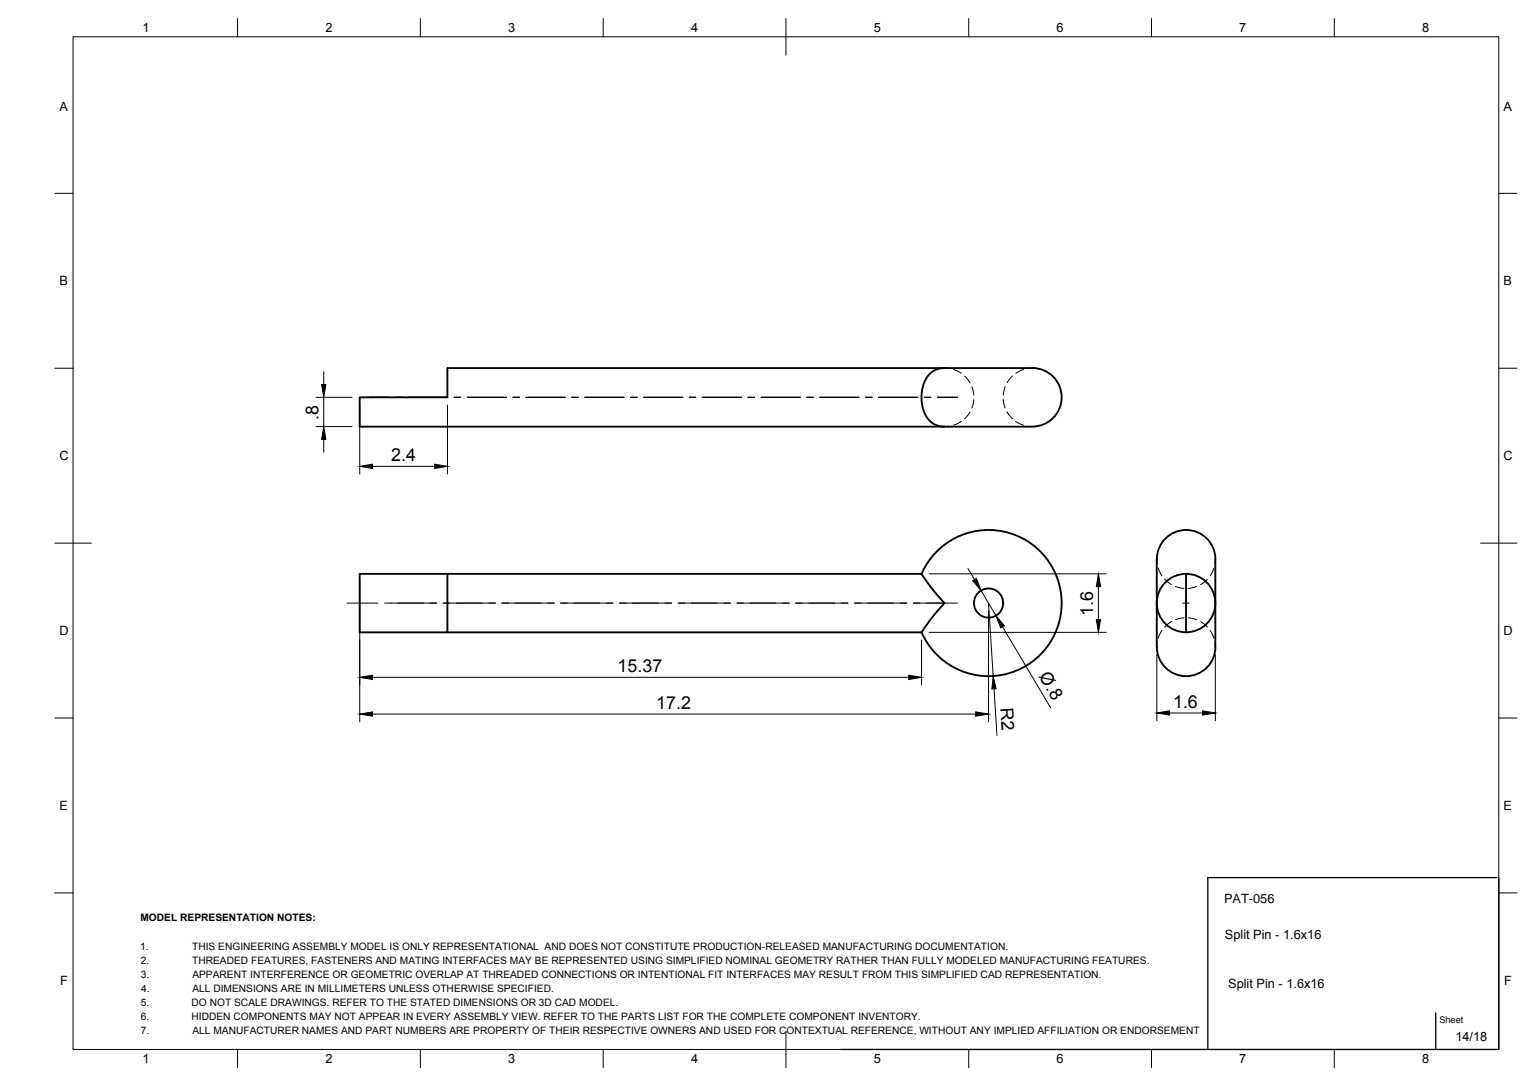
ISO-10303-21;
HEADER;
/* Generated by software containing ST-Developer
 * from STEP Tools, Inc. (www.steptools.com) 
 */

FILE_DESCRIPTION(
/* description */ ('Hook toggle clamp'),
/* implementation_level */ '2;1');

FILE_NAME(
/* name */ 'Split Pin - 1.6x16.step',
/* time_stamp */ '2026-10-27T21:56:56-07:00',
/* author */ (''),
/* organization */ (''),
/* preprocessor_version */ 'ST-DEVELOPER v20.2',
/* originating_system */ 'Autodesk Translation Framework v15.17.0.0',
/* authorisation */ '');

FILE_SCHEMA (('AUTOMOTIVE_DESIGN { 1 0 10303 214 3 1 1 }'));
ENDSEC;

DATA;
#10=MECHANICAL_DESIGN_GEOMETRIC_PRESENTATION_REPRESENTATION('',(#202),#5458);
#11=TOROIDAL_SURFACE('',#3441,0.12,0.08);
#17=B_SPLINE_CURVE_WITH_KNOTS('',3,(#5209,#5210,#5211,#5212,#5213,#5214,
#5215,#5216,#5217,#5218,#5219,#5220,#5221,#5222,#5223,#5224,#5225,#5226,
#5227,#5228,#5229,#5230,#5231,#5232,#5233,#5234),.UNSPECIFIED.,.F.,.F.,
(4,2,2,2,2,2,2,2,2,2,2,2,4),(-0.00054581412719389,0.,0.0281583564005144,
0.0618496465371181,0.0905865724114538,0.120694112793616,0.144966158459363,
0.16923820412511,0.199345744507272,0.228082670381608,0.261773960518212,
0.289932316918681,0.290478131045882),.UNSPECIFIED.);
#18=B_SPLINE_CURVE_WITH_KNOTS('',3,(#5235,#5236,#5237,#5238,#5239,#5240,
#5241,#5242,#5243,#5244,#5245,#5246,#5247,#5248,#5249,#5250,#5251,#5252,
#5253,#5254,#5255,#5256,#5257,#5258,#5259,#5260),.UNSPECIFIED.,.F.,.F.,
(4,2,2,2,2,2,2,2,2,2,2,2,4),(-0.000545814127196571,0.,0.0281583564006391,
0.0618496465374156,0.0905865724118984,0.120694112794215,0.144966158460086,
0.169238204125958,0.199345744508275,0.228082670382758,0.261773960519534,
0.289932316920171,0.29047813104737),.UNSPECIFIED.);
#168=SHAPE_REPRESENTATION_RELATIONSHIP('SRR','None',#5552,#185);
#185=ADVANCED_BREP_SHAPE_REPRESENTATION('',(#218),#5454);
#202=STYLED_ITEM('',(#5717),#218);
#218=MANIFOLD_SOLID_BREP('Body1',#2984);
#273=FACE_BOUND('',#766,.T.);
#378=PLANE('',#3444);
#379=PLANE('',#3446);
#380=PLANE('',#3450);
#541=FACE_OUTER_BOUND('',#765,.T.);
#542=FACE_OUTER_BOUND('',#767,.T.);
#543=FACE_OUTER_BOUND('',#768,.T.);
#544=FACE_OUTER_BOUND('',#769,.T.);
#545=FACE_OUTER_BOUND('',#770,.T.);
#765=EDGE_LOOP('',(#2645,#2646,#2647,#2648));
#766=EDGE_LOOP('',(#2649,#2650));
#767=EDGE_LOOP('',(#2651,#2652));
#768=EDGE_LOOP('',(#2653,#2654,#2655,#2656));
#769=EDGE_LOOP('',(#2657,#2658,#2659,#2660,#2661,#2662,#2663,#2664,#2665));
#770=EDGE_LOOP('',(#2666,#2667,#2668));
#1014=LINE('',#5265,#1251);
#1015=LINE('',#5268,#1252);
#1016=LINE('',#5270,#1253);
#1017=LINE('',#5271,#1254);
#1018=LINE('',#5275,#1255);
#1251=VECTOR('',#4270,1.);
#1252=VECTOR('',#4273,1.);
#1253=VECTOR('',#4274,1.);
#1254=VECTOR('',#4275,1.);
#1255=VECTOR('',#4280,0.08);
#1362=CIRCLE('',#3442,0.08);
#1363=CIRCLE('',#3443,0.04);
#1364=CIRCLE('',#3445,0.08);
#1365=CIRCLE('',#3448,0.08);
#1366=CIRCLE('',#3449,0.08);
#1593=VERTEX_POINT('',#5204);
#1594=VERTEX_POINT('',#5207);
#1595=VERTEX_POINT('',#5208);
#1596=VERTEX_POINT('',#5262);
#1597=VERTEX_POINT('',#5263);
#1598=VERTEX_POINT('',#5267);
#1599=VERTEX_POINT('',#5269);
#1600=VERTEX_POINT('',#5273);
#1949=EDGE_CURVE('',#1593,#1593,#1362,.T.);
#1950=EDGE_CURVE('',#1593,#1593,#1363,.T.);
#1951=EDGE_CURVE('',#1594,#1595,#17,.T.);
#1952=EDGE_CURVE('',#1595,#1594,#18,.T.);
#1953=EDGE_CURVE('',#1596,#1597,#1364,.T.);
#1954=EDGE_CURVE('',#1596,#1597,#1014,.T.);
#1955=EDGE_CURVE('',#1597,#1598,#1015,.T.);
#1956=EDGE_CURVE('',#1599,#1598,#1016,.T.);
#1957=EDGE_CURVE('',#1596,#1599,#1017,.T.);
#1958=EDGE_CURVE('',#1600,#1599,#1365,.T.);
#1959=EDGE_CURVE('',#1600,#1595,#1018,.T.);
#1960=EDGE_CURVE('',#1598,#1600,#1366,.T.);
#2645=ORIENTED_EDGE('',*,*,#1949,.F.);
#2646=ORIENTED_EDGE('',*,*,#1950,.T.);
#2647=ORIENTED_EDGE('',*,*,#1949,.T.);
#2648=ORIENTED_EDGE('',*,*,#1950,.F.);
#2649=ORIENTED_EDGE('',*,*,#1951,.F.);
#2650=ORIENTED_EDGE('',*,*,#1952,.F.);
#2651=ORIENTED_EDGE('',*,*,#1953,.T.);
#2652=ORIENTED_EDGE('',*,*,#1954,.F.);
#2653=ORIENTED_EDGE('',*,*,#1954,.T.);
#2654=ORIENTED_EDGE('',*,*,#1955,.T.);
#2655=ORIENTED_EDGE('',*,*,#1956,.F.);
#2656=ORIENTED_EDGE('',*,*,#1957,.F.);
#2657=ORIENTED_EDGE('',*,*,#1953,.F.);
#2658=ORIENTED_EDGE('',*,*,#1957,.T.);
#2659=ORIENTED_EDGE('',*,*,#1958,.F.);
#2660=ORIENTED_EDGE('',*,*,#1959,.T.);
#2661=ORIENTED_EDGE('',*,*,#1952,.T.);
#2662=ORIENTED_EDGE('',*,*,#1951,.T.);
#2663=ORIENTED_EDGE('',*,*,#1959,.F.);
#2664=ORIENTED_EDGE('',*,*,#1960,.F.);
#2665=ORIENTED_EDGE('',*,*,#1955,.F.);
#2666=ORIENTED_EDGE('',*,*,#1960,.T.);
#2667=ORIENTED_EDGE('',*,*,#1958,.T.);
#2668=ORIENTED_EDGE('',*,*,#1956,.T.);
#2791=CYLINDRICAL_SURFACE('',#3447,0.08);
#2945=ADVANCED_FACE('',(#541,#273),#11,.T.);
#2946=ADVANCED_FACE('',(#542),#378,.F.);
#2947=ADVANCED_FACE('',(#543),#379,.T.);
#2948=ADVANCED_FACE('',(#544),#2791,.T.);
#2949=ADVANCED_FACE('',(#545),#380,.F.);
#2984=CLOSED_SHELL('',(#2945,#2946,#2947,#2948,#2949));
#3440=AXIS2_PLACEMENT_3D('',#5202,#4258,#4259);
#3441=AXIS2_PLACEMENT_3D('',#5203,#4260,#4261);
#3442=AXIS2_PLACEMENT_3D('',#5205,#4262,#4263);
#3443=AXIS2_PLACEMENT_3D('',#5206,#4264,#4265);
#3444=AXIS2_PLACEMENT_3D('',#5261,#4266,#4267);
#3445=AXIS2_PLACEMENT_3D('',#5264,#4268,#4269);
#3446=AXIS2_PLACEMENT_3D('',#5266,#4271,#4272);
#3447=AXIS2_PLACEMENT_3D('',#5272,#4276,#4277);
#3448=AXIS2_PLACEMENT_3D('',#5274,#4278,#4279);
#3449=AXIS2_PLACEMENT_3D('',#5276,#4281,#4282);
#3450=AXIS2_PLACEMENT_3D('',#5277,#4283,#4284);
#4258=DIRECTION('axis',(0.,0.,1.));
#4259=DIRECTION('refdir',(1.,0.,0.));
#4260=DIRECTION('center_axis',(-1.,0.,0.));
#4261=DIRECTION('ref_axis',(0.,0.,1.));
#4262=DIRECTION('center_axis',(0.,-1.,1.38777878078145E-16));
#4263=DIRECTION('ref_axis',(0.,-1.38777878078145E-16,-1.));
#4264=DIRECTION('center_axis',(1.,0.,0.));
#4265=DIRECTION('ref_axis',(0.,0.,1.));
#4266=DIRECTION('center_axis',(0.,1.,0.));
#4267=DIRECTION('ref_axis',(1.,0.,0.));
#4268=DIRECTION('center_axis',(0.,-1.,0.));
#4269=DIRECTION('ref_axis',(1.,0.,0.));
#4270=DIRECTION('',(0.,0.,1.));
#4271=DIRECTION('center_axis',(1.,0.,0.));
#4272=DIRECTION('ref_axis',(0.,0.,1.));
#4273=DIRECTION('',(0.,-1.,0.));
#4274=DIRECTION('',(0.,0.,1.));
#4275=DIRECTION('',(0.,-1.,0.));
#4276=DIRECTION('center_axis',(0.,-1.,0.));
#4277=DIRECTION('ref_axis',(1.,0.,0.));
#4278=DIRECTION('center_axis',(0.,-1.,0.));
#4279=DIRECTION('ref_axis',(1.,0.,0.));
#4280=DIRECTION('',(0.,1.,0.));
#4281=DIRECTION('center_axis',(0.,-1.,0.));
#4282=DIRECTION('ref_axis',(1.,0.,0.));
#4283=DIRECTION('center_axis',(0.,1.,0.));
#4284=DIRECTION('ref_axis',(1.,0.,0.));
#5202=CARTESIAN_POINT('',(0.,0.,0.));
#5203=CARTESIAN_POINT('Origin',(0.,0.12,0.));
#5204=CARTESIAN_POINT('',(-9.79717439317883E-18,0.12,-0.04));
#5205=CARTESIAN_POINT('Origin',(0.,0.12,-0.12));
#5206=CARTESIAN_POINT('Origin',(9.79717439317883E-18,0.12,0.));
#5207=CARTESIAN_POINT('',(0.08,-4.89858719658941E-18,7.34788079488412E-18));
#5208=CARTESIAN_POINT('',(-0.08,-4.89858719658941E-18,7.34788079488412E-18));
#5209=CARTESIAN_POINT('Ctrl Pts',(0.08,-4.89858719658941E-18,7.34788079488412E-18));
#5210=CARTESIAN_POINT('Ctrl Pts',(0.08,-0.00012864962353541,0.000128649623535413));
#5211=CARTESIAN_POINT('Ctrl Pts',(0.0799996896739287,-0.00025719571182076,
0.000257402596003253));
#5212=CARTESIAN_POINT('Ctrl Pts',(0.0799669711262291,-0.00701193164572964,
0.00703384588894362));
#5213=CARTESIAN_POINT('Ctrl Pts',(0.0791054994909294,-0.0133457972655825,
0.0139383126556792));
#5214=CARTESIAN_POINT('Ctrl Pts',(0.0749700088488058,-0.0265076530862524,
0.0292212026164895));
#5215=CARTESIAN_POINT('Ctrl Pts',(0.0712702072865517,-0.0331317062461458,
0.0375603420117568));
#5216=CARTESIAN_POINT('Ctrl Pts',(0.0612858949407667,-0.0440683985740427,
0.0520545604187517));
#5217=CARTESIAN_POINT('Ctrl Pts',(0.0555090276731744,-0.0485199197794574,
0.0582717815295611));
#5218=CARTESIAN_POINT('Ctrl Pts',(0.0412398082144208,-0.0561090538733877,
0.0691638397919718));
#5219=CARTESIAN_POINT('Ctrl Pts',(0.0327878980890048,-0.059089642483296,
0.0736229049587921));
#5220=CARTESIAN_POINT('Ctrl Pts',(0.0159233027310102,-0.0625179833270725,
0.0787936360751706));
#5221=CARTESIAN_POINT('Ctrl Pts',(0.00801661414593076,-0.0633030277982336,
0.08));
#5222=CARTESIAN_POINT('Ctrl Pts',(-0.00801661414593074,-0.0633030277982336,
0.08));
#5223=CARTESIAN_POINT('Ctrl Pts',(-0.0159233027310102,-0.0625179833270726,
0.0787936360751706));
#5224=CARTESIAN_POINT('Ctrl Pts',(-0.0327878980890049,-0.059089642483296,
0.0736229049587921));
#5225=CARTESIAN_POINT('Ctrl Pts',(-0.0412398082144209,-0.0561090538733877,
0.0691638397919717));
#5226=CARTESIAN_POINT('Ctrl Pts',(-0.0555090276731744,-0.0485199197794574,
0.0582717815295611));
#5227=CARTESIAN_POINT('Ctrl Pts',(-0.0612858949407667,-0.0440683985740427,
0.0520545604187517));
#5228=CARTESIAN_POINT('Ctrl Pts',(-0.0712702072865517,-0.0331317062461458,
0.0375603420117568));
#5229=CARTESIAN_POINT('Ctrl Pts',(-0.0749700088488058,-0.0265076530862524,
0.0292212026164895));
#5230=CARTESIAN_POINT('Ctrl Pts',(-0.0791054994909264,-0.0133457972655921,
0.0139383126556903));
#5231=CARTESIAN_POINT('Ctrl Pts',(-0.0799669711262287,-0.00701193164579759,
0.0070338458890125));
#5232=CARTESIAN_POINT('Ctrl Pts',(-0.0799996896739287,-0.000257195711817665,
0.000257402596000083));
#5233=CARTESIAN_POINT('Ctrl Pts',(-0.08,-0.000128649623538514,0.000128649623538516));
#5234=CARTESIAN_POINT('Ctrl Pts',(-0.08,-4.89858719658941E-18,7.34788079488412E-18));
#5235=CARTESIAN_POINT('Ctrl Pts',(-0.08,-4.89858719658941E-18,7.34788079488412E-18));
#5236=CARTESIAN_POINT('Ctrl Pts',(-0.08,-0.000128649623536042,-0.00012864962353603));
#5237=CARTESIAN_POINT('Ctrl Pts',(-0.0799996896739287,-0.000257195711820127,
-0.000257402596002604));
#5238=CARTESIAN_POINT('Ctrl Pts',(-0.0799669711262289,-0.0070119316457589,
-0.00703384588897312));
#5239=CARTESIAN_POINT('Ctrl Pts',(-0.0791054994909281,-0.0133457972655867,
-0.0139383126556841));
#5240=CARTESIAN_POINT('Ctrl Pts',(-0.0749700088488058,-0.0265076530862525,
-0.0292212026164896));
#5241=CARTESIAN_POINT('Ctrl Pts',(-0.0712702072865516,-0.0331317062461459,
-0.0375603420117568));
#5242=CARTESIAN_POINT('Ctrl Pts',(-0.0612858949407667,-0.0440683985740427,
-0.0520545604187517));
#5243=CARTESIAN_POINT('Ctrl Pts',(-0.0555090276731744,-0.0485199197794574,
-0.0582717815295611));
#5244=CARTESIAN_POINT('Ctrl Pts',(-0.0412398082144209,-0.0561090538733877,
-0.0691638397919717));
#5245=CARTESIAN_POINT('Ctrl Pts',(-0.0327878980890049,-0.059089642483296,
-0.0736229049587921));
#5246=CARTESIAN_POINT('Ctrl Pts',(-0.0159233027310101,-0.0625179833270725,
-0.0787936360751706));
#5247=CARTESIAN_POINT('Ctrl Pts',(-0.00801661414593069,-0.0633030277982336,
-0.08));
#5248=CARTESIAN_POINT('Ctrl Pts',(0.0080166141459307,-0.0633030277982336,
-0.08));
#5249=CARTESIAN_POINT('Ctrl Pts',(0.0159233027310101,-0.0625179833270725,
-0.0787936360751706));
#5250=CARTESIAN_POINT('Ctrl Pts',(0.0327878980890049,-0.0590896424832959,
-0.0736229049587921));
#5251=CARTESIAN_POINT('Ctrl Pts',(0.0412398082144209,-0.0561090538733877,
-0.0691638397919717));
#5252=CARTESIAN_POINT('Ctrl Pts',(0.0555090276731744,-0.0485199197794574,
-0.0582717815295611));
#5253=CARTESIAN_POINT('Ctrl Pts',(0.0612858949407666,-0.0440683985740428,
-0.0520545604187518));
#5254=CARTESIAN_POINT('Ctrl Pts',(0.0712702072865517,-0.0331317062461458,
-0.0375603420117568));
#5255=CARTESIAN_POINT('Ctrl Pts',(0.0749700088488058,-0.0265076530862524,
-0.0292212026164895));
#5256=CARTESIAN_POINT('Ctrl Pts',(0.079105499490928,-0.013345797265587,
-0.0139383126556845));
#5257=CARTESIAN_POINT('Ctrl Pts',(0.0799669711262289,-0.00701193164576148,
-0.00703384588897579));
#5258=CARTESIAN_POINT('Ctrl Pts',(0.0799996896739287,-0.000257195711819584,
-0.000257402596002039));
#5259=CARTESIAN_POINT('Ctrl Pts',(0.08,-0.000128649623536605,-0.000128649623536593));
#5260=CARTESIAN_POINT('Ctrl Pts',(0.08,-4.89858719658941E-18,7.34788079488412E-18));
#5261=CARTESIAN_POINT('Origin',(0.04,-1.36,0.));
#5262=CARTESIAN_POINT('',(0.,-1.36,-0.08));
#5263=CARTESIAN_POINT('',(0.,-1.36,0.08));
#5264=CARTESIAN_POINT('Origin',(0.,-1.36,0.));
#5265=CARTESIAN_POINT('',(0.,-1.36,-0.04));
#5266=CARTESIAN_POINT('Origin',(0.,0.,-0.08));
#5267=CARTESIAN_POINT('',(0.,-1.6,0.08));
#5268=CARTESIAN_POINT('',(0.,0.,0.08));
#5269=CARTESIAN_POINT('',(0.,-1.6,-0.08));
#5270=CARTESIAN_POINT('',(0.,-1.6,-0.09));
#5271=CARTESIAN_POINT('',(0.,0.,-0.08));
#5272=CARTESIAN_POINT('Origin',(0.,0.,0.));
#5273=CARTESIAN_POINT('',(-0.08,-1.6,-9.79717439317883E-18));
#5274=CARTESIAN_POINT('Origin',(0.,-1.6,0.));
#5275=CARTESIAN_POINT('',(-0.08,0.,-9.79717439317883E-18));
#5276=CARTESIAN_POINT('Origin',(0.,-1.6,0.));
#5277=CARTESIAN_POINT('Origin',(-0.04,-1.6,0.));
#5431=UNCERTAINTY_MEASURE_WITH_UNIT(LENGTH_MEASURE(0.001),#5459,
'DISTANCE_ACCURACY_VALUE',
'Maximum model space distance between geometric entities at asserted c
onnectivities');
#5435=UNCERTAINTY_MEASURE_WITH_UNIT(LENGTH_MEASURE(0.001),#5459,
'DISTANCE_ACCURACY_VALUE',
'Maximum model space distance between geometric entities at asserted c
onnectivities');
#5454=(
GEOMETRIC_REPRESENTATION_CONTEXT(3)
GLOBAL_UNCERTAINTY_ASSIGNED_CONTEXT((#5431))
GLOBAL_UNIT_ASSIGNED_CONTEXT((#5459,#5461,#5462))
REPRESENTATION_CONTEXT('','3D')
);
#5458=(
GEOMETRIC_REPRESENTATION_CONTEXT(3)
GLOBAL_UNCERTAINTY_ASSIGNED_CONTEXT((#5435))
GLOBAL_UNIT_ASSIGNED_CONTEXT((#5459,#5461,#5462))
REPRESENTATION_CONTEXT('','3D')
);
#5459=(
LENGTH_UNIT()
NAMED_UNIT(*)
SI_UNIT(.CENTI.,.METRE.)
);
#5461=(
NAMED_UNIT(*)
PLANE_ANGLE_UNIT()
SI_UNIT($,.RADIAN.)
);
#5462=(
NAMED_UNIT(*)
SI_UNIT($,.STERADIAN.)
SOLID_ANGLE_UNIT()
);
#5481=SHAPE_DEFINITION_REPRESENTATION(#5508,#5552);
#5508=PRODUCT_DEFINITION_SHAPE('',$,#5575);
#5552=SHAPE_REPRESENTATION('',(#3440),#5454);
#5556=PRODUCT_DEFINITION_CONTEXT('part definition',#5624,'design');
#5575=PRODUCT_DEFINITION('Split Pin - 1.6x16','Split Pin - 1.6x16',#5597,
#5556);
#5597=PRODUCT_DEFINITION_FORMATION('',$,#5644);
#5624=APPLICATION_CONTEXT(
'Core Data for Automotive Mechanical Design Process');
#5625=PRODUCT_CONTEXT('part definition',#5624,'mechanical');
#5644=PRODUCT('Split Pin - 1.6x16','Split Pin - 1.6x16',
'Split Pin - 1.6x16',(#5625));
#5711=COLOUR_RGB('Grey',0.48,0.52,0.57);
#5712=FILL_AREA_STYLE_COLOUR('',#5711);
#5713=FILL_AREA_STYLE('',(#5712));
#5714=SURFACE_STYLE_FILL_AREA(#5713);
#5715=SURFACE_SIDE_STYLE('',(#5714));
#5716=SURFACE_STYLE_USAGE(.BOTH.,#5715);
#5717=PRESENTATION_STYLE_ASSIGNMENT((#5716));
ENDSEC;
END-ISO-10303-21;
